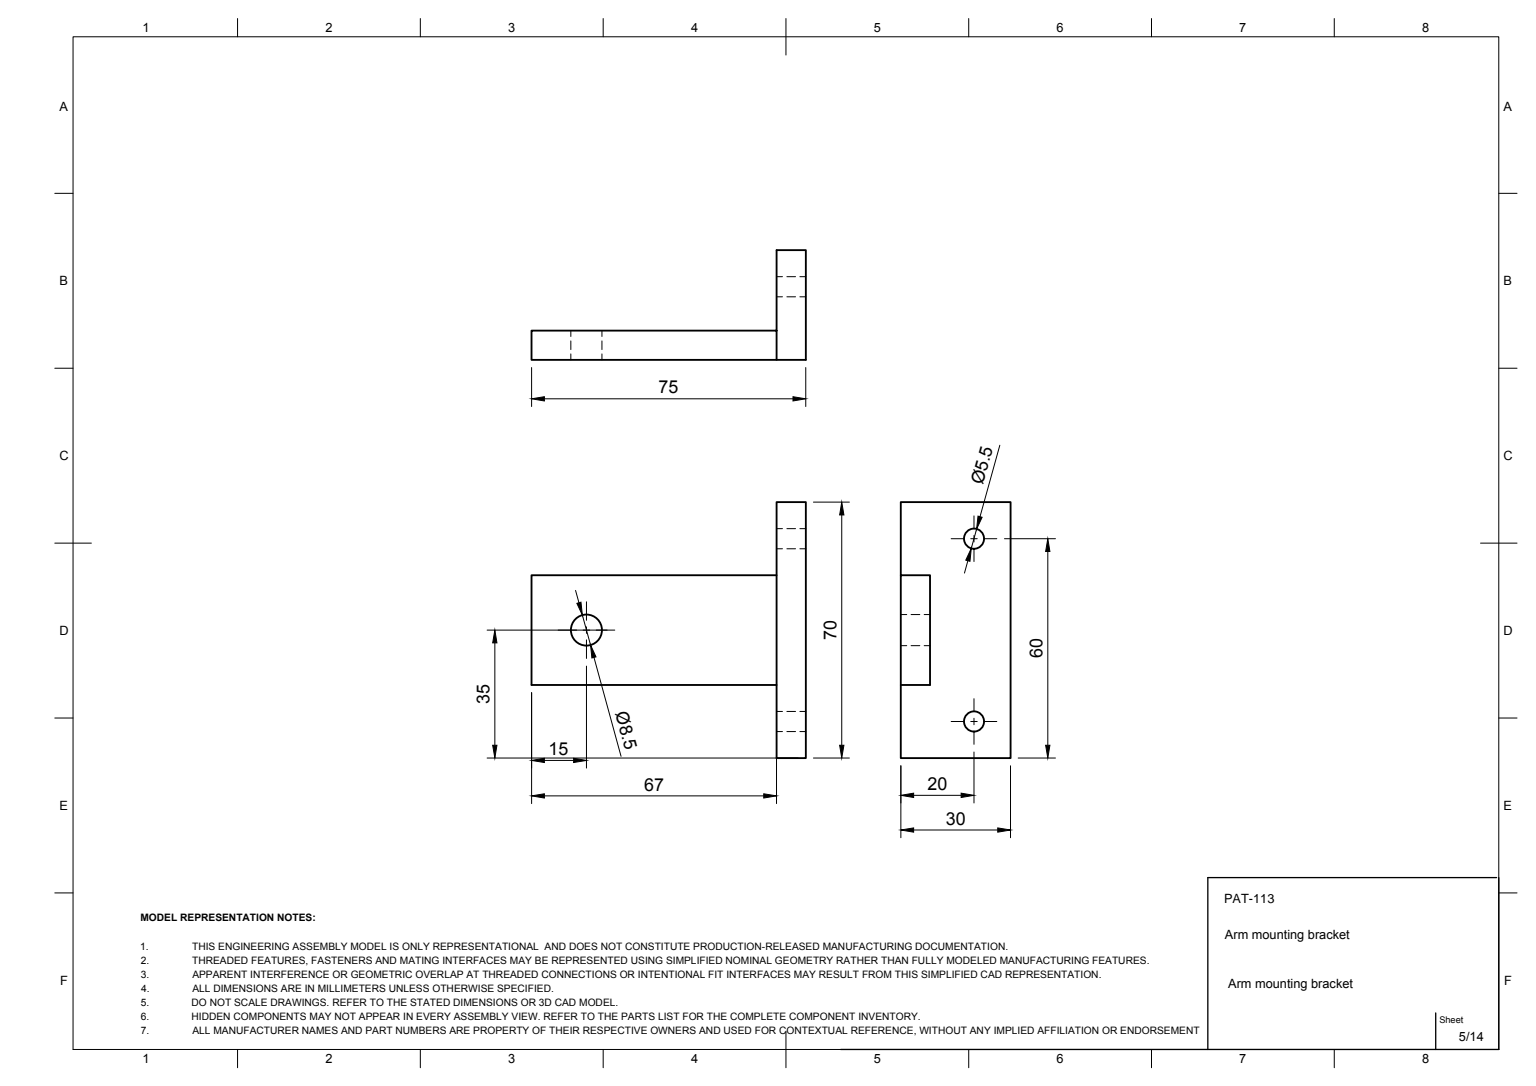
ISO-10303-21;
HEADER;
/* Generated by software containing ST-Developer
 * from STEP Tools, Inc. (www.steptools.com) 
 */

FILE_DESCRIPTION(
/* description */ ('Two-link friction support arm'),
/* implementation_level */ '2;1');

FILE_NAME(
/* name */ 'Arm mounting bracket.step',
/* time_stamp */ '2026-10-27T20:01:49-07:00',
/* author */ (''),
/* organization */ (''),
/* preprocessor_version */ 'ST-DEVELOPER v20.2',
/* originating_system */ 'Autodesk Translation Framework v15.17.0.0',
/* authorisation */ '');

FILE_SCHEMA (('AUTOMOTIVE_DESIGN { 1 0 10303 214 3 1 1 }'));
ENDSEC;

DATA;
#10=MECHANICAL_DESIGN_GEOMETRIC_PRESENTATION_REPRESENTATION('',(#195),#5492);
#173=SHAPE_REPRESENTATION_RELATIONSHIP('SRR','None',#5564,#184);
#184=ADVANCED_BREP_SHAPE_REPRESENTATION('',(#206),#5478);
#195=STYLED_ITEM('',(#5680),#206);
#206=MANIFOLD_SOLID_BREP('Body1',#3171);
#216=FACE_BOUND('',#547,.T.);
#217=FACE_BOUND('',#549,.T.);
#218=FACE_BOUND('',#550,.T.);
#219=FACE_BOUND('',#552,.T.);
#220=FACE_BOUND('',#557,.T.);
#221=FACE_BOUND('',#558,.T.);
#250=PLANE('',#3317);
#251=PLANE('',#3318);
#252=PLANE('',#3319);
#253=PLANE('',#3320);
#254=PLANE('',#3321);
#255=PLANE('',#3322);
#256=PLANE('',#3323);
#257=PLANE('',#3324);
#258=PLANE('',#3325);
#259=PLANE('',#3326);
#373=FACE_OUTER_BOUND('',#540,.T.);
#374=FACE_OUTER_BOUND('',#541,.T.);
#375=FACE_OUTER_BOUND('',#542,.T.);
#376=FACE_OUTER_BOUND('',#543,.T.);
#377=FACE_OUTER_BOUND('',#544,.T.);
#378=FACE_OUTER_BOUND('',#545,.T.);
#379=FACE_OUTER_BOUND('',#546,.T.);
#380=FACE_OUTER_BOUND('',#548,.T.);
#381=FACE_OUTER_BOUND('',#551,.T.);
#382=FACE_OUTER_BOUND('',#553,.T.);
#383=FACE_OUTER_BOUND('',#554,.T.);
#384=FACE_OUTER_BOUND('',#555,.T.);
#385=FACE_OUTER_BOUND('',#556,.T.);
#540=EDGE_LOOP('',(#2138,#2139,#2140,#2141));
#541=EDGE_LOOP('',(#2142,#2143,#2144,#2145));
#542=EDGE_LOOP('',(#2146,#2147,#2148,#2149));
#543=EDGE_LOOP('',(#2150,#2151,#2152,#2153));
#544=EDGE_LOOP('',(#2154,#2155,#2156,#2157));
#545=EDGE_LOOP('',(#2158,#2159,#2160,#2161));
#546=EDGE_LOOP('',(#2162,#2163,#2164,#2165));
#547=EDGE_LOOP('',(#2166));
#548=EDGE_LOOP('',(#2167,#2168,#2169,#2170,#2171,#2172,#2173,#2174));
#549=EDGE_LOOP('',(#2175));
#550=EDGE_LOOP('',(#2176));
#551=EDGE_LOOP('',(#2177,#2178,#2179,#2180,#2181,#2182,#2183,#2184));
#552=EDGE_LOOP('',(#2185));
#553=EDGE_LOOP('',(#2186,#2187,#2188,#2189));
#554=EDGE_LOOP('',(#2190,#2191,#2192,#2193));
#555=EDGE_LOOP('',(#2194,#2195,#2196,#2197));
#556=EDGE_LOOP('',(#2198,#2199,#2200,#2201));
#557=EDGE_LOOP('',(#2202));
#558=EDGE_LOOP('',(#2203));
#741=LINE('',#4525,#1054);
#742=LINE('',#4531,#1055);
#743=LINE('',#4537,#1056);
#744=LINE('',#4542,#1057);
#745=LINE('',#4544,#1058);
#746=LINE('',#4546,#1059);
#747=LINE('',#4547,#1060);
#748=LINE('',#4551,#1061);
#749=LINE('',#4553,#1062);
#750=LINE('',#4555,#1063);
#751=LINE('',#4556,#1064);
#752=LINE('',#4558,#1065);
#753=LINE('',#4559,#1066);
#754=LINE('',#4561,#1067);
#755=LINE('',#4564,#1068);
#756=LINE('',#4566,#1069);
#757=LINE('',#4568,#1070);
#758=LINE('',#4570,#1071);
#759=LINE('',#4571,#1072);
#760=LINE('',#4575,#1073);
#761=LINE('',#4576,#1074);
#762=LINE('',#4577,#1075);
#763=LINE('',#4580,#1076);
#764=LINE('',#4581,#1077);
#765=LINE('',#4584,#1078);
#766=LINE('',#4585,#1079);
#767=LINE('',#4587,#1080);
#1054=VECTOR('',#3615,0.275);
#1055=VECTOR('',#3622,0.275);
#1056=VECTOR('',#3629,0.425);
#1057=VECTOR('',#3634,1.);
#1058=VECTOR('',#3635,1.);
#1059=VECTOR('',#3636,1.);
#1060=VECTOR('',#3637,1.);
#1061=VECTOR('',#3640,1.);
#1062=VECTOR('',#3641,1.);
#1063=VECTOR('',#3642,1.);
#1064=VECTOR('',#3643,1.);
#1065=VECTOR('',#3646,1.);
#1066=VECTOR('',#3647,1.);
#1067=VECTOR('',#3650,1.);
#1068=VECTOR('',#3653,1.);
#1069=VECTOR('',#3654,1.);
#1070=VECTOR('',#3655,1.);
#1071=VECTOR('',#3656,1.);
#1072=VECTOR('',#3657,1.);
#1073=VECTOR('',#3660,1.);
#1074=VECTOR('',#3661,1.);
#1075=VECTOR('',#3662,1.);
#1076=VECTOR('',#3665,1.);
#1077=VECTOR('',#3666,1.);
#1078=VECTOR('',#3669,1.);
#1079=VECTOR('',#3670,1.);
#1080=VECTOR('',#3673,1.);
#1367=CIRCLE('',#3309,0.275);
#1368=CIRCLE('',#3310,0.275);
#1369=CIRCLE('',#3312,0.275);
#1370=CIRCLE('',#3313,0.275);
#1371=CIRCLE('',#3315,0.425);
#1372=CIRCLE('',#3316,0.425);
#1449=VERTEX_POINT('',#4522);
#1450=VERTEX_POINT('',#4524);
#1451=VERTEX_POINT('',#4528);
#1452=VERTEX_POINT('',#4530);
#1453=VERTEX_POINT('',#4534);
#1454=VERTEX_POINT('',#4536);
#1455=VERTEX_POINT('',#4540);
#1456=VERTEX_POINT('',#4541);
#1457=VERTEX_POINT('',#4543);
#1458=VERTEX_POINT('',#4545);
#1459=VERTEX_POINT('',#4549);
#1460=VERTEX_POINT('',#4550);
#1461=VERTEX_POINT('',#4552);
#1462=VERTEX_POINT('',#4554);
#1463=VERTEX_POINT('',#4563);
#1464=VERTEX_POINT('',#4565);
#1465=VERTEX_POINT('',#4567);
#1466=VERTEX_POINT('',#4569);
#1467=VERTEX_POINT('',#4573);
#1468=VERTEX_POINT('',#4574);
#1469=VERTEX_POINT('',#4579);
#1470=VERTEX_POINT('',#4583);
#1723=EDGE_CURVE('',#1449,#1449,#1367,.T.);
#1724=EDGE_CURVE('',#1449,#1450,#741,.T.);
#1725=EDGE_CURVE('',#1450,#1450,#1368,.T.);
#1726=EDGE_CURVE('',#1451,#1451,#1369,.T.);
#1727=EDGE_CURVE('',#1451,#1452,#742,.T.);
#1728=EDGE_CURVE('',#1452,#1452,#1370,.T.);
#1729=EDGE_CURVE('',#1453,#1453,#1371,.T.);
#1730=EDGE_CURVE('',#1453,#1454,#743,.T.);
#1731=EDGE_CURVE('',#1454,#1454,#1372,.T.);
#1732=EDGE_CURVE('',#1455,#1456,#744,.T.);
#1733=EDGE_CURVE('',#1455,#1457,#745,.T.);
#1734=EDGE_CURVE('',#1458,#1457,#746,.T.);
#1735=EDGE_CURVE('',#1456,#1458,#747,.T.);
#1736=EDGE_CURVE('',#1459,#1460,#748,.T.);
#1737=EDGE_CURVE('',#1461,#1459,#749,.T.);
#1738=EDGE_CURVE('',#1462,#1461,#750,.T.);
#1739=EDGE_CURVE('',#1460,#1462,#751,.T.);
#1740=EDGE_CURVE('',#1460,#1455,#752,.T.);
#1741=EDGE_CURVE('',#1457,#1462,#753,.T.);
#1742=EDGE_CURVE('',#1459,#1456,#754,.T.);
#1743=EDGE_CURVE('',#1458,#1463,#755,.T.);
#1744=EDGE_CURVE('',#1463,#1464,#756,.T.);
#1745=EDGE_CURVE('',#1464,#1465,#757,.T.);
#1746=EDGE_CURVE('',#1465,#1466,#758,.T.);
#1747=EDGE_CURVE('',#1466,#1461,#759,.T.);
#1748=EDGE_CURVE('',#1467,#1468,#760,.T.);
#1749=EDGE_CURVE('',#1468,#1463,#761,.T.);
#1750=EDGE_CURVE('',#1467,#1466,#762,.T.);
#1751=EDGE_CURVE('',#1469,#1467,#763,.T.);
#1752=EDGE_CURVE('',#1469,#1465,#764,.T.);
#1753=EDGE_CURVE('',#1470,#1469,#765,.T.);
#1754=EDGE_CURVE('',#1470,#1464,#766,.T.);
#1755=EDGE_CURVE('',#1468,#1470,#767,.T.);
#2138=ORIENTED_EDGE('',*,*,#1723,.F.);
#2139=ORIENTED_EDGE('',*,*,#1724,.T.);
#2140=ORIENTED_EDGE('',*,*,#1725,.F.);
#2141=ORIENTED_EDGE('',*,*,#1724,.F.);
#2142=ORIENTED_EDGE('',*,*,#1726,.F.);
#2143=ORIENTED_EDGE('',*,*,#1727,.T.);
#2144=ORIENTED_EDGE('',*,*,#1728,.F.);
#2145=ORIENTED_EDGE('',*,*,#1727,.F.);
#2146=ORIENTED_EDGE('',*,*,#1729,.F.);
#2147=ORIENTED_EDGE('',*,*,#1730,.T.);
#2148=ORIENTED_EDGE('',*,*,#1731,.F.);
#2149=ORIENTED_EDGE('',*,*,#1730,.F.);
#2150=ORIENTED_EDGE('',*,*,#1732,.F.);
#2151=ORIENTED_EDGE('',*,*,#1733,.T.);
#2152=ORIENTED_EDGE('',*,*,#1734,.F.);
#2153=ORIENTED_EDGE('',*,*,#1735,.F.);
#2154=ORIENTED_EDGE('',*,*,#1736,.F.);
#2155=ORIENTED_EDGE('',*,*,#1737,.F.);
#2156=ORIENTED_EDGE('',*,*,#1738,.F.);
#2157=ORIENTED_EDGE('',*,*,#1739,.F.);
#2158=ORIENTED_EDGE('',*,*,#1740,.F.);
#2159=ORIENTED_EDGE('',*,*,#1739,.T.);
#2160=ORIENTED_EDGE('',*,*,#1741,.F.);
#2161=ORIENTED_EDGE('',*,*,#1733,.F.);
#2162=ORIENTED_EDGE('',*,*,#1740,.T.);
#2163=ORIENTED_EDGE('',*,*,#1732,.T.);
#2164=ORIENTED_EDGE('',*,*,#1742,.F.);
#2165=ORIENTED_EDGE('',*,*,#1736,.T.);
#2166=ORIENTED_EDGE('',*,*,#1729,.T.);
#2167=ORIENTED_EDGE('',*,*,#1737,.T.);
#2168=ORIENTED_EDGE('',*,*,#1742,.T.);
#2169=ORIENTED_EDGE('',*,*,#1735,.T.);
#2170=ORIENTED_EDGE('',*,*,#1743,.T.);
#2171=ORIENTED_EDGE('',*,*,#1744,.T.);
#2172=ORIENTED_EDGE('',*,*,#1745,.T.);
#2173=ORIENTED_EDGE('',*,*,#1746,.T.);
#2174=ORIENTED_EDGE('',*,*,#1747,.T.);
#2175=ORIENTED_EDGE('',*,*,#1725,.T.);
#2176=ORIENTED_EDGE('',*,*,#1728,.T.);
#2177=ORIENTED_EDGE('',*,*,#1748,.T.);
#2178=ORIENTED_EDGE('',*,*,#1749,.T.);
#2179=ORIENTED_EDGE('',*,*,#1743,.F.);
#2180=ORIENTED_EDGE('',*,*,#1734,.T.);
#2181=ORIENTED_EDGE('',*,*,#1741,.T.);
#2182=ORIENTED_EDGE('',*,*,#1738,.T.);
#2183=ORIENTED_EDGE('',*,*,#1747,.F.);
#2184=ORIENTED_EDGE('',*,*,#1750,.F.);
#2185=ORIENTED_EDGE('',*,*,#1731,.T.);
#2186=ORIENTED_EDGE('',*,*,#1751,.T.);
#2187=ORIENTED_EDGE('',*,*,#1750,.T.);
#2188=ORIENTED_EDGE('',*,*,#1746,.F.);
#2189=ORIENTED_EDGE('',*,*,#1752,.F.);
#2190=ORIENTED_EDGE('',*,*,#1753,.T.);
#2191=ORIENTED_EDGE('',*,*,#1752,.T.);
#2192=ORIENTED_EDGE('',*,*,#1745,.F.);
#2193=ORIENTED_EDGE('',*,*,#1754,.F.);
#2194=ORIENTED_EDGE('',*,*,#1755,.T.);
#2195=ORIENTED_EDGE('',*,*,#1754,.T.);
#2196=ORIENTED_EDGE('',*,*,#1744,.F.);
#2197=ORIENTED_EDGE('',*,*,#1749,.F.);
#2198=ORIENTED_EDGE('',*,*,#1755,.F.);
#2199=ORIENTED_EDGE('',*,*,#1748,.F.);
#2200=ORIENTED_EDGE('',*,*,#1751,.F.);
#2201=ORIENTED_EDGE('',*,*,#1753,.F.);
#2202=ORIENTED_EDGE('',*,*,#1723,.T.);
#2203=ORIENTED_EDGE('',*,*,#1726,.T.);
#2968=CYLINDRICAL_SURFACE('',#3308,0.275);
#2969=CYLINDRICAL_SURFACE('',#3311,0.275);
#2970=CYLINDRICAL_SURFACE('',#3314,0.425);
#3004=ADVANCED_FACE('',(#373),#2968,.F.);
#3005=ADVANCED_FACE('',(#374),#2969,.F.);
#3006=ADVANCED_FACE('',(#375),#2970,.F.);
#3007=ADVANCED_FACE('',(#376),#250,.T.);
#3008=ADVANCED_FACE('',(#377),#251,.T.);
#3009=ADVANCED_FACE('',(#378),#252,.T.);
#3010=ADVANCED_FACE('',(#379,#216),#253,.F.);
#3011=ADVANCED_FACE('',(#380,#217,#218),#254,.T.);
#3012=ADVANCED_FACE('',(#381,#219),#255,.T.);
#3013=ADVANCED_FACE('',(#382),#256,.T.);
#3014=ADVANCED_FACE('',(#383),#257,.T.);
#3015=ADVANCED_FACE('',(#384),#258,.T.);
#3016=ADVANCED_FACE('',(#385,#220,#221),#259,.F.);
#3171=CLOSED_SHELL('',(#3004,#3005,#3006,#3007,#3008,#3009,#3010,#3011,
#3012,#3013,#3014,#3015,#3016));
#3307=AXIS2_PLACEMENT_3D('',#4520,#3609,#3610);
#3308=AXIS2_PLACEMENT_3D('',#4521,#3611,#3612);
#3309=AXIS2_PLACEMENT_3D('',#4523,#3613,#3614);
#3310=AXIS2_PLACEMENT_3D('',#4526,#3616,#3617);
#3311=AXIS2_PLACEMENT_3D('',#4527,#3618,#3619);
#3312=AXIS2_PLACEMENT_3D('',#4529,#3620,#3621);
#3313=AXIS2_PLACEMENT_3D('',#4532,#3623,#3624);
#3314=AXIS2_PLACEMENT_3D('',#4533,#3625,#3626);
#3315=AXIS2_PLACEMENT_3D('',#4535,#3627,#3628);
#3316=AXIS2_PLACEMENT_3D('',#4538,#3630,#3631);
#3317=AXIS2_PLACEMENT_3D('',#4539,#3632,#3633);
#3318=AXIS2_PLACEMENT_3D('',#4548,#3638,#3639);
#3319=AXIS2_PLACEMENT_3D('',#4557,#3644,#3645);
#3320=AXIS2_PLACEMENT_3D('',#4560,#3648,#3649);
#3321=AXIS2_PLACEMENT_3D('',#4562,#3651,#3652);
#3322=AXIS2_PLACEMENT_3D('',#4572,#3658,#3659);
#3323=AXIS2_PLACEMENT_3D('',#4578,#3663,#3664);
#3324=AXIS2_PLACEMENT_3D('',#4582,#3667,#3668);
#3325=AXIS2_PLACEMENT_3D('',#4586,#3671,#3672);
#3326=AXIS2_PLACEMENT_3D('',#4588,#3674,#3675);
#3609=DIRECTION('axis',(0.,0.,1.));
#3610=DIRECTION('refdir',(1.,0.,0.));
#3611=DIRECTION('center_axis',(0.,0.,1.));
#3612=DIRECTION('ref_axis',(1.,0.,0.));
#3613=DIRECTION('center_axis',(0.,0.,1.));
#3614=DIRECTION('ref_axis',(1.,0.,0.));
#3615=DIRECTION('',(0.,0.,1.));
#3616=DIRECTION('center_axis',(0.,0.,-1.));
#3617=DIRECTION('ref_axis',(1.,0.,0.));
#3618=DIRECTION('center_axis',(0.,0.,1.));
#3619=DIRECTION('ref_axis',(1.,0.,0.));
#3620=DIRECTION('center_axis',(0.,0.,1.));
#3621=DIRECTION('ref_axis',(1.,0.,0.));
#3622=DIRECTION('',(0.,0.,1.));
#3623=DIRECTION('center_axis',(0.,0.,-1.));
#3624=DIRECTION('ref_axis',(1.,0.,0.));
#3625=DIRECTION('center_axis',(0.,1.,0.));
#3626=DIRECTION('ref_axis',(1.,0.,0.));
#3627=DIRECTION('center_axis',(0.,1.,0.));
#3628=DIRECTION('ref_axis',(1.,0.,0.));
#3629=DIRECTION('',(0.,1.,0.));
#3630=DIRECTION('center_axis',(0.,-1.,0.));
#3631=DIRECTION('ref_axis',(1.,0.,0.));
#3632=DIRECTION('center_axis',(-1.,0.,0.));
#3633=DIRECTION('ref_axis',(0.,0.,1.));
#3634=DIRECTION('',(0.,0.,-1.));
#3635=DIRECTION('',(0.,1.,0.));
#3636=DIRECTION('',(0.,0.,1.));
#3637=DIRECTION('',(0.,1.,0.));
#3638=DIRECTION('center_axis',(1.,0.,0.));
#3639=DIRECTION('ref_axis',(0.,0.,-1.));
#3640=DIRECTION('',(0.,0.,1.));
#3641=DIRECTION('',(0.,-1.,0.));
#3642=DIRECTION('',(0.,0.,-1.));
#3643=DIRECTION('',(0.,1.,0.));
#3644=DIRECTION('center_axis',(0.,0.,1.));
#3645=DIRECTION('ref_axis',(1.,0.,0.));
#3646=DIRECTION('',(-1.,0.,0.));
#3647=DIRECTION('',(1.,0.,0.));
#3648=DIRECTION('center_axis',(0.,1.,0.));
#3649=DIRECTION('ref_axis',(1.,0.,0.));
#3650=DIRECTION('',(-1.,0.,0.));
#3651=DIRECTION('center_axis',(0.,0.,1.));
#3652=DIRECTION('ref_axis',(1.,0.,0.));
#3653=DIRECTION('',(-1.,0.,0.));
#3654=DIRECTION('',(0.,-1.,0.));
#3655=DIRECTION('',(1.,0.,0.));
#3656=DIRECTION('',(0.,1.,0.));
#3657=DIRECTION('',(-1.,0.,0.));
#3658=DIRECTION('center_axis',(0.,1.,0.));
#3659=DIRECTION('ref_axis',(-1.,0.,0.));
#3660=DIRECTION('',(-1.,0.,0.));
#3661=DIRECTION('',(0.,0.,1.));
#3662=DIRECTION('',(0.,0.,1.));
#3663=DIRECTION('center_axis',(1.,0.,0.));
#3664=DIRECTION('ref_axis',(0.,1.,0.));
#3665=DIRECTION('',(0.,1.,0.));
#3666=DIRECTION('',(0.,0.,1.));
#3667=DIRECTION('center_axis',(0.,-1.,0.));
#3668=DIRECTION('ref_axis',(1.,0.,0.));
#3669=DIRECTION('',(1.,0.,0.));
#3670=DIRECTION('',(0.,0.,1.));
#3671=DIRECTION('center_axis',(-1.,0.,0.));
#3672=DIRECTION('ref_axis',(0.,-1.,0.));
#3673=DIRECTION('',(0.,-1.,0.));
#3674=DIRECTION('center_axis',(0.,0.,1.));
#3675=DIRECTION('ref_axis',(1.,0.,0.));
#4520=CARTESIAN_POINT('',(0.,0.,0.));
#4521=CARTESIAN_POINT('Origin',(2.5,-2.,1.9));
#4522=CARTESIAN_POINT('',(2.225,-2.,2.));
#4523=CARTESIAN_POINT('Origin',(2.5,-2.,2.));
#4524=CARTESIAN_POINT('',(2.225,-2.,2.8));
#4525=CARTESIAN_POINT('',(2.225,-2.,1.9));
#4526=CARTESIAN_POINT('Origin',(2.5,-2.,2.8));
#4527=CARTESIAN_POINT('Origin',(7.5,-2.,1.9));
#4528=CARTESIAN_POINT('',(7.225,-2.,2.));
#4529=CARTESIAN_POINT('Origin',(7.5,-2.,2.));
#4530=CARTESIAN_POINT('',(7.225,-2.,2.8));
#4531=CARTESIAN_POINT('',(7.225,-2.,1.9));
#4532=CARTESIAN_POINT('Origin',(7.5,-2.,2.8));
#4533=CARTESIAN_POINT('Origin',(5.,-0.9,8.));
#4534=CARTESIAN_POINT('',(4.575,-0.8,8.));
#4535=CARTESIAN_POINT('Origin',(5.,-0.8,8.));
#4536=CARTESIAN_POINT('',(4.575,0.,8.));
#4537=CARTESIAN_POINT('',(4.575,-0.9,8.));
#4538=CARTESIAN_POINT('Origin',(5.,0.,8.));
#4539=CARTESIAN_POINT('Origin',(3.5,-0.8,2.8));
#4540=CARTESIAN_POINT('',(3.5,-0.8,9.5));
#4541=CARTESIAN_POINT('',(3.5,-0.8,2.8));
#4542=CARTESIAN_POINT('',(3.5,-0.8,9.5));
#4543=CARTESIAN_POINT('',(3.5,0.,9.5));
#4544=CARTESIAN_POINT('',(3.5,-0.8,9.5));
#4545=CARTESIAN_POINT('',(3.5,0.,2.8));
#4546=CARTESIAN_POINT('',(3.5,0.,9.5));
#4547=CARTESIAN_POINT('',(3.5,-1.15,2.8));
#4548=CARTESIAN_POINT('Origin',(6.5,-0.8,9.5));
#4549=CARTESIAN_POINT('',(6.5,-0.8,2.8));
#4550=CARTESIAN_POINT('',(6.5,-0.8,9.5));
#4551=CARTESIAN_POINT('',(6.5,-0.8,2.8));
#4552=CARTESIAN_POINT('',(6.5,0.,2.8));
#4553=CARTESIAN_POINT('',(6.5,-1.15,2.8));
#4554=CARTESIAN_POINT('',(6.5,0.,9.5));
#4555=CARTESIAN_POINT('',(6.5,0.,2.8));
#4556=CARTESIAN_POINT('',(6.5,-0.8,9.5));
#4557=CARTESIAN_POINT('Origin',(3.5,-0.8,9.5));
#4558=CARTESIAN_POINT('',(6.5,-0.8,9.5));
#4559=CARTESIAN_POINT('',(6.5,0.,9.5));
#4560=CARTESIAN_POINT('Origin',(5.,-0.8,6.15));
#4561=CARTESIAN_POINT('',(5.,-0.8,2.8));
#4562=CARTESIAN_POINT('Origin',(5.,-1.5,2.8));
#4563=CARTESIAN_POINT('',(1.5,0.,2.8));
#4564=CARTESIAN_POINT('',(8.5,0.,2.8));
#4565=CARTESIAN_POINT('',(1.5,-3.,2.8));
#4566=CARTESIAN_POINT('',(1.5,0.,2.8));
#4567=CARTESIAN_POINT('',(8.5,-3.,2.8));
#4568=CARTESIAN_POINT('',(1.5,-3.,2.8));
#4569=CARTESIAN_POINT('',(8.5,0.,2.8));
#4570=CARTESIAN_POINT('',(8.5,-3.,2.8));
#4571=CARTESIAN_POINT('',(8.5,0.,2.8));
#4572=CARTESIAN_POINT('Origin',(8.5,0.,2.));
#4573=CARTESIAN_POINT('',(8.5,0.,2.));
#4574=CARTESIAN_POINT('',(1.5,0.,2.));
#4575=CARTESIAN_POINT('',(8.5,0.,2.));
#4576=CARTESIAN_POINT('',(1.5,0.,2.));
#4577=CARTESIAN_POINT('',(8.5,0.,2.));
#4578=CARTESIAN_POINT('Origin',(8.5,-3.,2.));
#4579=CARTESIAN_POINT('',(8.5,-3.,2.));
#4580=CARTESIAN_POINT('',(8.5,-3.,2.));
#4581=CARTESIAN_POINT('',(8.5,-3.,2.));
#4582=CARTESIAN_POINT('Origin',(1.5,-3.,2.));
#4583=CARTESIAN_POINT('',(1.5,-3.,2.));
#4584=CARTESIAN_POINT('',(1.5,-3.,2.));
#4585=CARTESIAN_POINT('',(1.5,-3.,2.));
#4586=CARTESIAN_POINT('Origin',(1.5,0.,2.));
#4587=CARTESIAN_POINT('',(1.5,0.,2.));
#4588=CARTESIAN_POINT('Origin',(5.,-1.5,2.));
#5461=UNCERTAINTY_MEASURE_WITH_UNIT(LENGTH_MEASURE(0.001),#5493,
'DISTANCE_ACCURACY_VALUE',
'Maximum model space distance between geometric entities at asserted c
onnectivities');
#5475=UNCERTAINTY_MEASURE_WITH_UNIT(LENGTH_MEASURE(0.001),#5493,
'DISTANCE_ACCURACY_VALUE',
'Maximum model space distance between geometric entities at asserted c
onnectivities');
#5478=(
GEOMETRIC_REPRESENTATION_CONTEXT(3)
GLOBAL_UNCERTAINTY_ASSIGNED_CONTEXT((#5461))
GLOBAL_UNIT_ASSIGNED_CONTEXT((#5493,#5495,#5496))
REPRESENTATION_CONTEXT('','3D')
);
#5492=(
GEOMETRIC_REPRESENTATION_CONTEXT(3)
GLOBAL_UNCERTAINTY_ASSIGNED_CONTEXT((#5475))
GLOBAL_UNIT_ASSIGNED_CONTEXT((#5493,#5495,#5496))
REPRESENTATION_CONTEXT('','3D')
);
#5493=(
LENGTH_UNIT()
NAMED_UNIT(*)
SI_UNIT(.CENTI.,.METRE.)
);
#5495=(
NAMED_UNIT(*)
PLANE_ANGLE_UNIT()
SI_UNIT($,.RADIAN.)
);
#5496=(
NAMED_UNIT(*)
SI_UNIT($,.STERADIAN.)
SOLID_ANGLE_UNIT()
);
#5499=SHAPE_DEFINITION_REPRESENTATION(#5515,#5564);
#5515=PRODUCT_DEFINITION_SHAPE('',$,#5581);
#5564=SHAPE_REPRESENTATION('',(#3307),#5478);
#5578=PRODUCT_DEFINITION_CONTEXT('part definition',#5628,'design');
#5581=PRODUCT_DEFINITION('Arm mounting bracket','Arm mounting bracket',
#5597,#5578);
#5597=PRODUCT_DEFINITION_FORMATION('',$,#5632);
#5628=APPLICATION_CONTEXT(
'Core Data for Automotive Mechanical Design Process');
#5629=PRODUCT_CONTEXT('part definition',#5628,'mechanical');
#5632=PRODUCT('Arm mounting bracket','Arm mounting bracket',
'Arm mounting bracket',(#5629));
#5674=COLOUR_RGB('Dark Blue',0.08,0.2,0.34);
#5675=FILL_AREA_STYLE_COLOUR('',#5674);
#5676=FILL_AREA_STYLE('',(#5675));
#5677=SURFACE_STYLE_FILL_AREA(#5676);
#5678=SURFACE_SIDE_STYLE('',(#5677));
#5679=SURFACE_STYLE_USAGE(.BOTH.,#5678);
#5680=PRESENTATION_STYLE_ASSIGNMENT((#5679));
ENDSEC;
END-ISO-10303-21;
